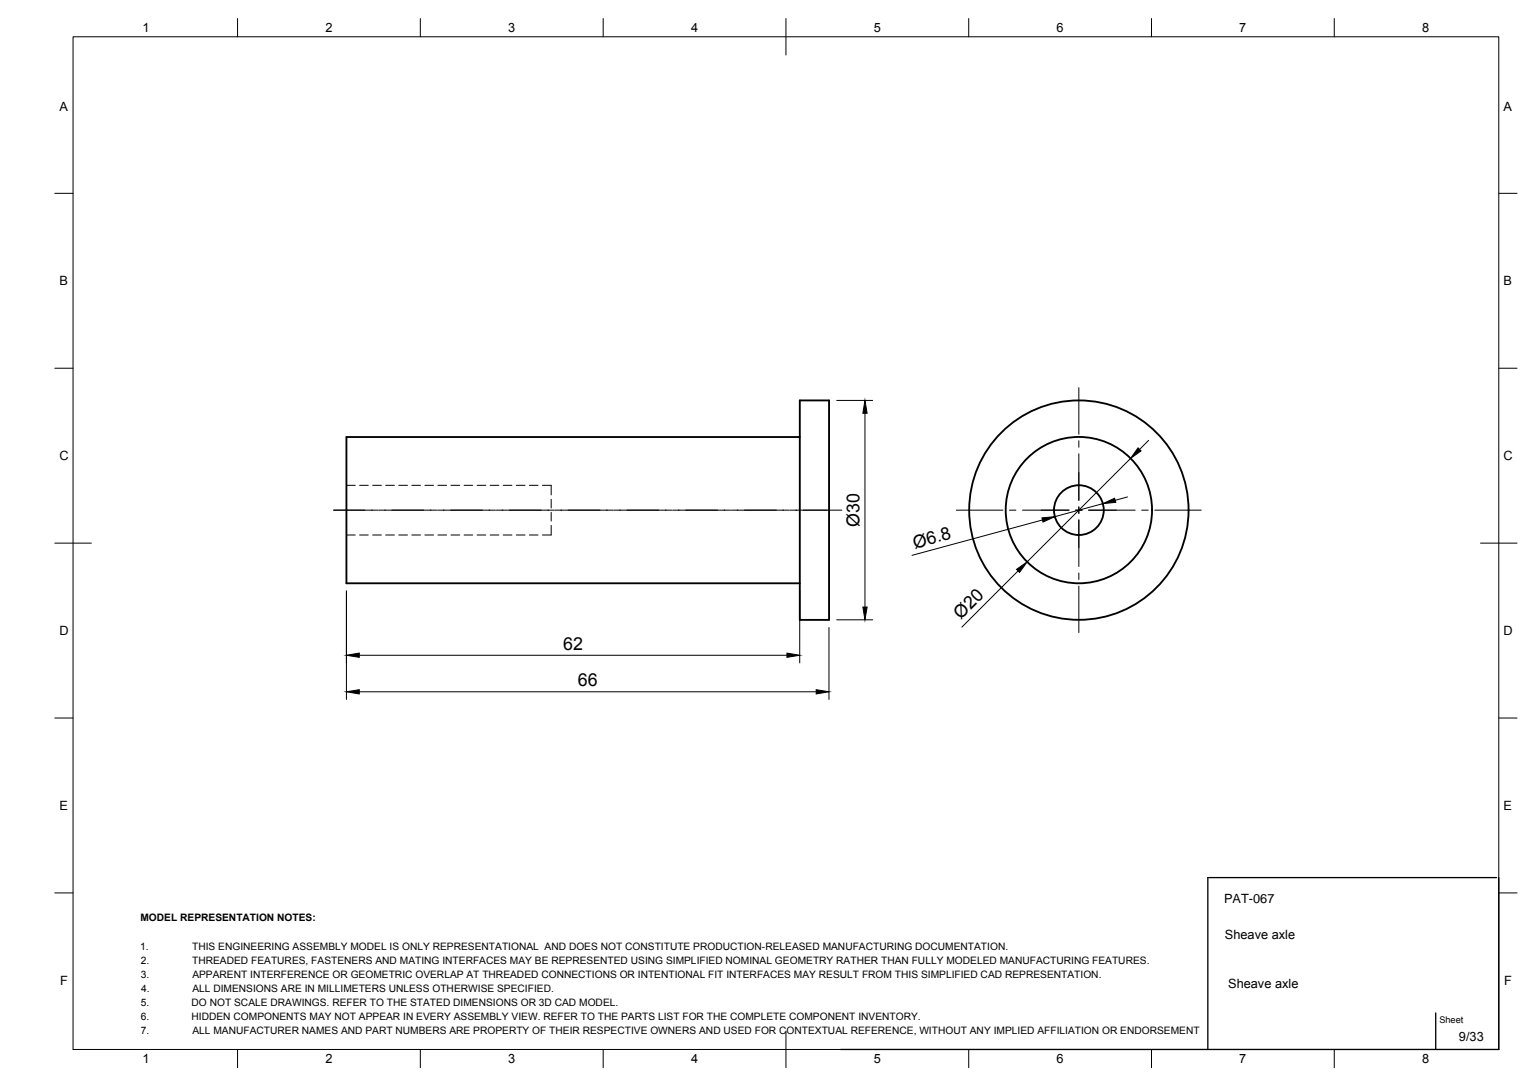
ISO-10303-21;
HEADER;
/* Generated by software containing ST-Developer
 * from STEP Tools, Inc. (www.steptools.com) 
 */

FILE_DESCRIPTION(
/* description */ ('Lifting hook block with sheave'),
/* implementation_level */ '2;1');

FILE_NAME(
/* name */ 'Sheave axle.step',
/* time_stamp */ '2026-10-28T03:23:54-07:00',
/* author */ (''),
/* organization */ (''),
/* preprocessor_version */ 'ST-DEVELOPER v20.2',
/* originating_system */ 'Autodesk Translation Framework v15.17.0.0',
/* authorisation */ '');

FILE_SCHEMA (('AUTOMOTIVE_DESIGN { 1 0 10303 214 3 1 1 }'));
ENDSEC;

DATA;
#10=MECHANICAL_DESIGN_GEOMETRIC_PRESENTATION_REPRESENTATION('',(#355),#9391);
#295=SHAPE_REPRESENTATION_RELATIONSHIP('SRR','None',#9526,#325);
#325=ADVANCED_BREP_SHAPE_REPRESENTATION('',(#393),#9361);
#355=STYLED_ITEM('',(#9759),#393);
#393=MANIFOLD_SOLID_BREP('Body1',#4891);
#523=LINE('',#7926,#811);
#524=LINE('',#7936,#812);
#525=LINE('',#7942,#813);
#811=VECTOR('',#6328,0.34);
#812=VECTOR('',#6341,1.5);
#813=VECTOR('',#6350,1.);
#1031=CYLINDRICAL_SURFACE('',#5407,0.34);
#1032=CYLINDRICAL_SURFACE('',#5414,1.5);
#1033=CYLINDRICAL_SURFACE('',#5417,1.);
#1143=FACE_BOUND('',#1613,.T.);
#1144=FACE_BOUND('',#1618,.T.);
#1285=FACE_OUTER_BOUND('',#1610,.T.);
#1286=FACE_OUTER_BOUND('',#1611,.T.);
#1287=FACE_OUTER_BOUND('',#1612,.T.);
#1288=FACE_OUTER_BOUND('',#1614,.T.);
#1289=FACE_OUTER_BOUND('',#1615,.T.);
#1290=FACE_OUTER_BOUND('',#1616,.T.);
#1291=FACE_OUTER_BOUND('',#1617,.T.);
#1610=EDGE_LOOP('',(#3584,#3585,#3586,#3587));
#1611=EDGE_LOOP('',(#3588));
#1612=EDGE_LOOP('',(#3589));
#1613=EDGE_LOOP('',(#3590));
#1614=EDGE_LOOP('',(#3591,#3592,#3593,#3594));
#1615=EDGE_LOOP('',(#3595));
#1616=EDGE_LOOP('',(#3596,#3597,#3598,#3599));
#1617=EDGE_LOOP('',(#3600));
#1618=EDGE_LOOP('',(#3601));
#1993=CIRCLE('',#5408,0.34);
#1994=CIRCLE('',#5409,0.34);
#1995=CIRCLE('',#5412,1.5);
#1996=CIRCLE('',#5413,1.);
#1997=CIRCLE('',#5415,1.5);
#1998=CIRCLE('',#5418,1.);
#2326=VERTEX_POINT('',#7923);
#2327=VERTEX_POINT('',#7925);
#2328=VERTEX_POINT('',#7930);
#2329=VERTEX_POINT('',#7932);
#2330=VERTEX_POINT('',#7935);
#2331=VERTEX_POINT('',#7940);
#2796=EDGE_CURVE('',#2326,#2326,#1993,.T.);
#2797=EDGE_CURVE('',#2326,#2327,#523,.T.);
#2798=EDGE_CURVE('',#2327,#2327,#1994,.T.);
#2799=EDGE_CURVE('',#2328,#2328,#1995,.T.);
#2800=EDGE_CURVE('',#2329,#2329,#1996,.T.);
#2801=EDGE_CURVE('',#2328,#2330,#524,.T.);
#2802=EDGE_CURVE('',#2330,#2330,#1997,.T.);
#2803=EDGE_CURVE('',#2331,#2331,#1998,.T.);
#2804=EDGE_CURVE('',#2331,#2329,#525,.T.);
#3584=ORIENTED_EDGE('',*,*,#2796,.F.);
#3585=ORIENTED_EDGE('',*,*,#2797,.T.);
#3586=ORIENTED_EDGE('',*,*,#2798,.F.);
#3587=ORIENTED_EDGE('',*,*,#2797,.F.);
#3588=ORIENTED_EDGE('',*,*,#2796,.T.);
#3589=ORIENTED_EDGE('',*,*,#2799,.T.);
#3590=ORIENTED_EDGE('',*,*,#2800,.F.);
#3591=ORIENTED_EDGE('',*,*,#2799,.F.);
#3592=ORIENTED_EDGE('',*,*,#2801,.T.);
#3593=ORIENTED_EDGE('',*,*,#2802,.T.);
#3594=ORIENTED_EDGE('',*,*,#2801,.F.);
#3595=ORIENTED_EDGE('',*,*,#2802,.F.);
#3596=ORIENTED_EDGE('',*,*,#2803,.F.);
#3597=ORIENTED_EDGE('',*,*,#2804,.T.);
#3598=ORIENTED_EDGE('',*,*,#2800,.T.);
#3599=ORIENTED_EDGE('',*,*,#2804,.F.);
#3600=ORIENTED_EDGE('',*,*,#2803,.T.);
#3601=ORIENTED_EDGE('',*,*,#2798,.T.);
#4484=PLANE('',#5410);
#4485=PLANE('',#5411);
#4486=PLANE('',#5416);
#4487=PLANE('',#5419);
#4661=ADVANCED_FACE('',(#1285),#1031,.F.);
#4662=ADVANCED_FACE('',(#1286),#4484,.T.);
#4663=ADVANCED_FACE('',(#1287,#1143),#4485,.T.);
#4664=ADVANCED_FACE('',(#1288),#1032,.T.);
#4665=ADVANCED_FACE('',(#1289),#4486,.F.);
#4666=ADVANCED_FACE('',(#1290),#1033,.T.);
#4667=ADVANCED_FACE('',(#1291,#1144),#4487,.T.);
#4891=CLOSED_SHELL('',(#4661,#4662,#4663,#4664,#4665,#4666,#4667));
#5406=AXIS2_PLACEMENT_3D('',#7921,#6322,#6323);
#5407=AXIS2_PLACEMENT_3D('',#7922,#6324,#6325);
#5408=AXIS2_PLACEMENT_3D('',#7924,#6326,#6327);
#5409=AXIS2_PLACEMENT_3D('',#7927,#6329,#6330);
#5410=AXIS2_PLACEMENT_3D('',#7928,#6331,#6332);
#5411=AXIS2_PLACEMENT_3D('',#7929,#6333,#6334);
#5412=AXIS2_PLACEMENT_3D('',#7931,#6335,#6336);
#5413=AXIS2_PLACEMENT_3D('',#7933,#6337,#6338);
#5414=AXIS2_PLACEMENT_3D('',#7934,#6339,#6340);
#5415=AXIS2_PLACEMENT_3D('',#7937,#6342,#6343);
#5416=AXIS2_PLACEMENT_3D('',#7938,#6344,#6345);
#5417=AXIS2_PLACEMENT_3D('',#7939,#6346,#6347);
#5418=AXIS2_PLACEMENT_3D('',#7941,#6348,#6349);
#5419=AXIS2_PLACEMENT_3D('',#7943,#6351,#6352);
#6322=DIRECTION('axis',(0.,0.,1.));
#6323=DIRECTION('refdir',(1.,0.,0.));
#6324=DIRECTION('center_axis',(0.,1.,0.));
#6325=DIRECTION('ref_axis',(1.,0.,0.));
#6326=DIRECTION('center_axis',(0.,1.,0.));
#6327=DIRECTION('ref_axis',(1.,0.,0.));
#6328=DIRECTION('',(0.,1.,0.));
#6329=DIRECTION('center_axis',(0.,-1.,0.));
#6330=DIRECTION('ref_axis',(1.,0.,0.));
#6331=DIRECTION('center_axis',(0.,1.,0.));
#6332=DIRECTION('ref_axis',(1.,0.,0.));
#6333=DIRECTION('center_axis',(0.,1.,0.));
#6334=DIRECTION('ref_axis',(1.,0.,0.));
#6335=DIRECTION('center_axis',(0.,1.,0.));
#6336=DIRECTION('ref_axis',(1.,0.,0.));
#6337=DIRECTION('center_axis',(0.,1.,0.));
#6338=DIRECTION('ref_axis',(1.,0.,0.));
#6339=DIRECTION('center_axis',(0.,1.,0.));
#6340=DIRECTION('ref_axis',(1.,0.,0.));
#6341=DIRECTION('',(0.,-1.,0.));
#6342=DIRECTION('center_axis',(0.,1.,0.));
#6343=DIRECTION('ref_axis',(1.,0.,0.));
#6344=DIRECTION('center_axis',(0.,1.,0.));
#6345=DIRECTION('ref_axis',(1.,0.,0.));
#6346=DIRECTION('center_axis',(0.,1.,0.));
#6347=DIRECTION('ref_axis',(1.,0.,0.));
#6348=DIRECTION('center_axis',(0.,1.,0.));
#6349=DIRECTION('ref_axis',(1.,0.,0.));
#6350=DIRECTION('',(0.,-1.,0.));
#6351=DIRECTION('center_axis',(0.,1.,0.));
#6352=DIRECTION('ref_axis',(1.,0.,0.));
#7921=CARTESIAN_POINT('',(0.,0.,0.));
#7922=CARTESIAN_POINT('Origin',(0.,0.3,12.));
#7923=CARTESIAN_POINT('',(-0.34,0.3,12.));
#7924=CARTESIAN_POINT('Origin',(0.,0.3,12.));
#7925=CARTESIAN_POINT('',(-0.34,3.1,12.));
#7926=CARTESIAN_POINT('',(-0.34,0.3,12.));
#7927=CARTESIAN_POINT('Origin',(0.,3.1,12.));
#7928=CARTESIAN_POINT('Origin',(0.,0.3,12.));
#7929=CARTESIAN_POINT('Origin',(0.,-3.1,12.));
#7930=CARTESIAN_POINT('',(-1.5,-3.1,12.));
#7931=CARTESIAN_POINT('Origin',(0.,-3.1,12.));
#7932=CARTESIAN_POINT('',(-1.,-3.1,12.));
#7933=CARTESIAN_POINT('Origin',(0.,-3.1,12.));
#7934=CARTESIAN_POINT('Origin',(0.,-3.5,12.));
#7935=CARTESIAN_POINT('',(-1.5,-3.5,12.));
#7936=CARTESIAN_POINT('',(-1.5,-3.5,12.));
#7937=CARTESIAN_POINT('Origin',(0.,-3.5,12.));
#7938=CARTESIAN_POINT('Origin',(0.,-3.5,12.));
#7939=CARTESIAN_POINT('Origin',(0.,-3.1,12.));
#7940=CARTESIAN_POINT('',(-1.,3.1,12.));
#7941=CARTESIAN_POINT('Origin',(0.,3.1,12.));
#7942=CARTESIAN_POINT('',(-1.,-3.1,12.));
#7943=CARTESIAN_POINT('Origin',(0.,3.1,12.));
#9324=UNCERTAINTY_MEASURE_WITH_UNIT(LENGTH_MEASURE(0.001),#9392,
'DISTANCE_ACCURACY_VALUE',
'Maximum model space distance between geometric entities at asserted c
onnectivities');
#9354=UNCERTAINTY_MEASURE_WITH_UNIT(LENGTH_MEASURE(0.001),#9392,
'DISTANCE_ACCURACY_VALUE',
'Maximum model space distance between geometric entities at asserted c
onnectivities');
#9361=(
GEOMETRIC_REPRESENTATION_CONTEXT(3)
GLOBAL_UNCERTAINTY_ASSIGNED_CONTEXT((#9324))
GLOBAL_UNIT_ASSIGNED_CONTEXT((#9392,#9394,#9395))
REPRESENTATION_CONTEXT('','3D')
);
#9391=(
GEOMETRIC_REPRESENTATION_CONTEXT(3)
GLOBAL_UNCERTAINTY_ASSIGNED_CONTEXT((#9354))
GLOBAL_UNIT_ASSIGNED_CONTEXT((#9392,#9394,#9395))
REPRESENTATION_CONTEXT('','3D')
);
#9392=(
LENGTH_UNIT()
NAMED_UNIT(*)
SI_UNIT(.CENTI.,.METRE.)
);
#9394=(
NAMED_UNIT(*)
PLANE_ANGLE_UNIT()
SI_UNIT($,.RADIAN.)
);
#9395=(
NAMED_UNIT(*)
SI_UNIT($,.STERADIAN.)
SOLID_ANGLE_UNIT()
);
#9402=SHAPE_DEFINITION_REPRESENTATION(#9438,#9526);
#9438=PRODUCT_DEFINITION_SHAPE('',$,#9563);
#9526=SHAPE_REPRESENTATION('',(#5406),#9361);
#9556=PRODUCT_DEFINITION_CONTEXT('part definition',#9666,'design');
#9563=PRODUCT_DEFINITION('Sheave axle','Sheave axle',#9599,#9556);
#9599=PRODUCT_DEFINITION_FORMATION('',$,#9674);
#9666=APPLICATION_CONTEXT(
'Core Data for Automotive Mechanical Design Process');
#9667=PRODUCT_CONTEXT('part definition',#9666,'mechanical');
#9674=PRODUCT('Sheave axle','Sheave axle','Sheave axle',(#9667));
#9753=COLOUR_RGB('Grey',0.48,0.52,0.57);
#9754=FILL_AREA_STYLE_COLOUR('',#9753);
#9755=FILL_AREA_STYLE('',(#9754));
#9756=SURFACE_STYLE_FILL_AREA(#9755);
#9757=SURFACE_SIDE_STYLE('',(#9756));
#9758=SURFACE_STYLE_USAGE(.BOTH.,#9757);
#9759=PRESENTATION_STYLE_ASSIGNMENT((#9758));
ENDSEC;
END-ISO-10303-21;
